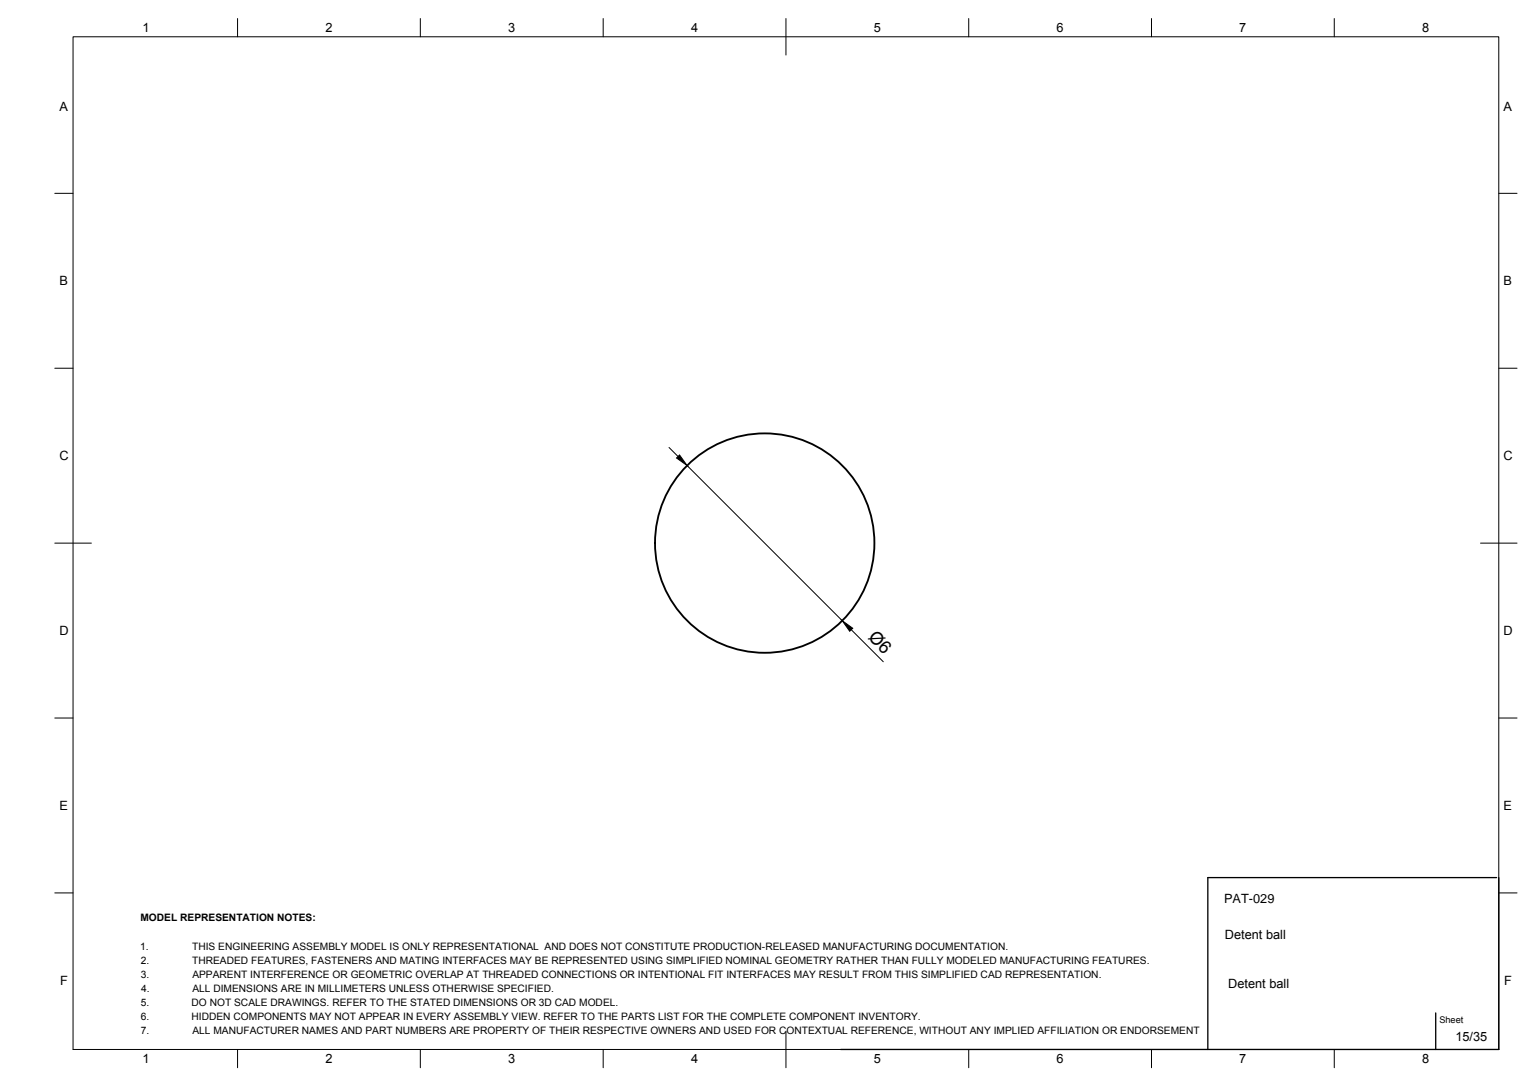
ISO-10303-21;
HEADER;
/* Generated by software containing ST-Developer
 * from STEP Tools, Inc. (www.steptools.com) 
 */

FILE_DESCRIPTION(
/* description */ ('Door-style hinge test fixture with detent'),
/* implementation_level */ '2;1');

FILE_NAME(
/* name */ 'Detent ball.step',
/* time_stamp */ '2026-10-28T03:24:57-07:00',
/* author */ (''),
/* organization */ (''),
/* preprocessor_version */ 'ST-DEVELOPER v20.2',
/* originating_system */ 'Autodesk Translation Framework v15.17.0.0',
/* authorisation */ '');

FILE_SCHEMA (('AUTOMOTIVE_DESIGN { 1 0 10303 214 3 1 1 }'));
ENDSEC;

DATA;
#10=MECHANICAL_DESIGN_GEOMETRIC_PRESENTATION_REPRESENTATION('',(#333),#9813);
#242=SPHERICAL_SURFACE('',#5356,0.3);
#270=SHAPE_REPRESENTATION_RELATIONSHIP('SRR','None',#9947,#301);
#301=ADVANCED_BREP_SHAPE_REPRESENTATION('',(#373),#9790);
#333=STYLED_ITEM('',(#10197),#373);
#373=MANIFOLD_SOLID_BREP('Body1',#4764);
#774=FACE_OUTER_BOUND('',#1119,.T.);
#1119=EDGE_LOOP('',(#3729,#3730));
#2068=CIRCLE('',#5357,0.3);
#2395=VERTEX_POINT('',#7857);
#2396=VERTEX_POINT('',#7858);
#2881=EDGE_CURVE('',#2395,#2396,#2068,.T.);
#3729=ORIENTED_EDGE('',*,*,#2881,.T.);
#3730=ORIENTED_EDGE('',*,*,#2881,.F.);
#4579=ADVANCED_FACE('',(#774),#242,.T.);
#4764=CLOSED_SHELL('',(#4579));
#5355=AXIS2_PLACEMENT_3D('',#7855,#6352,#6353);
#5356=AXIS2_PLACEMENT_3D('',#7856,#6354,#6355);
#5357=AXIS2_PLACEMENT_3D('',#7859,#6356,#6357);
#6352=DIRECTION('axis',(0.,0.,1.));
#6353=DIRECTION('refdir',(1.,0.,0.));
#6354=DIRECTION('center_axis',(6.12323399573677E-17,0.,1.));
#6355=DIRECTION('ref_axis',(1.,0.,0.));
#6356=DIRECTION('center_axis',(0.,-1.,0.));
#6357=DIRECTION('ref_axis',(-1.,0.,0.));
#7855=CARTESIAN_POINT('',(0.,0.,0.));
#7856=CARTESIAN_POINT('Origin',(0.,-2.13,7.2));
#7857=CARTESIAN_POINT('',(-1.83697019872103E-17,-2.13,7.5));
#7858=CARTESIAN_POINT('',(-1.83697019872103E-17,-2.13,6.9));
#7859=CARTESIAN_POINT('Origin',(0.,-2.13,7.2));
#9754=UNCERTAINTY_MEASURE_WITH_UNIT(LENGTH_MEASURE(0.001),#9814,
'DISTANCE_ACCURACY_VALUE',
'Maximum model space distance between geometric entities at asserted c
onnectivities');
#9777=UNCERTAINTY_MEASURE_WITH_UNIT(LENGTH_MEASURE(0.001),#9814,
'DISTANCE_ACCURACY_VALUE',
'Maximum model space distance between geometric entities at asserted c
onnectivities');
#9790=(
GEOMETRIC_REPRESENTATION_CONTEXT(3)
GLOBAL_UNCERTAINTY_ASSIGNED_CONTEXT((#9754))
GLOBAL_UNIT_ASSIGNED_CONTEXT((#9814,#9816,#9817))
REPRESENTATION_CONTEXT('','3D')
);
#9813=(
GEOMETRIC_REPRESENTATION_CONTEXT(3)
GLOBAL_UNCERTAINTY_ASSIGNED_CONTEXT((#9777))
GLOBAL_UNIT_ASSIGNED_CONTEXT((#9814,#9816,#9817))
REPRESENTATION_CONTEXT('','3D')
);
#9814=(
LENGTH_UNIT()
NAMED_UNIT(*)
SI_UNIT(.CENTI.,.METRE.)
);
#9816=(
NAMED_UNIT(*)
PLANE_ANGLE_UNIT()
SI_UNIT($,.RADIAN.)
);
#9817=(
NAMED_UNIT(*)
SI_UNIT($,.STERADIAN.)
SOLID_ANGLE_UNIT()
);
#9830=SHAPE_DEFINITION_REPRESENTATION(#9865,#9947);
#9865=PRODUCT_DEFINITION_SHAPE('',$,#9983);
#9947=SHAPE_REPRESENTATION('',(#5355),#9790);
#9970=PRODUCT_DEFINITION_CONTEXT('part definition',#10077,'design');
#9983=PRODUCT_DEFINITION('Detent ball','Detent ball',#10018,#9970);
#10018=PRODUCT_DEFINITION_FORMATION('',$,#10091);
#10077=APPLICATION_CONTEXT(
'Core Data for Automotive Mechanical Design Process');
#10078=PRODUCT_CONTEXT('part definition',#10077,'mechanical');
#10091=PRODUCT('Detent ball','Detent ball','Detent ball',(#10078));
#10191=COLOUR_RGB('Off White',0.89,0.88,0.83);
#10192=FILL_AREA_STYLE_COLOUR('',#10191);
#10193=FILL_AREA_STYLE('',(#10192));
#10194=SURFACE_STYLE_FILL_AREA(#10193);
#10195=SURFACE_SIDE_STYLE('',(#10194));
#10196=SURFACE_STYLE_USAGE(.BOTH.,#10195);
#10197=PRESENTATION_STYLE_ASSIGNMENT((#10196));
ENDSEC;
END-ISO-10303-21;
